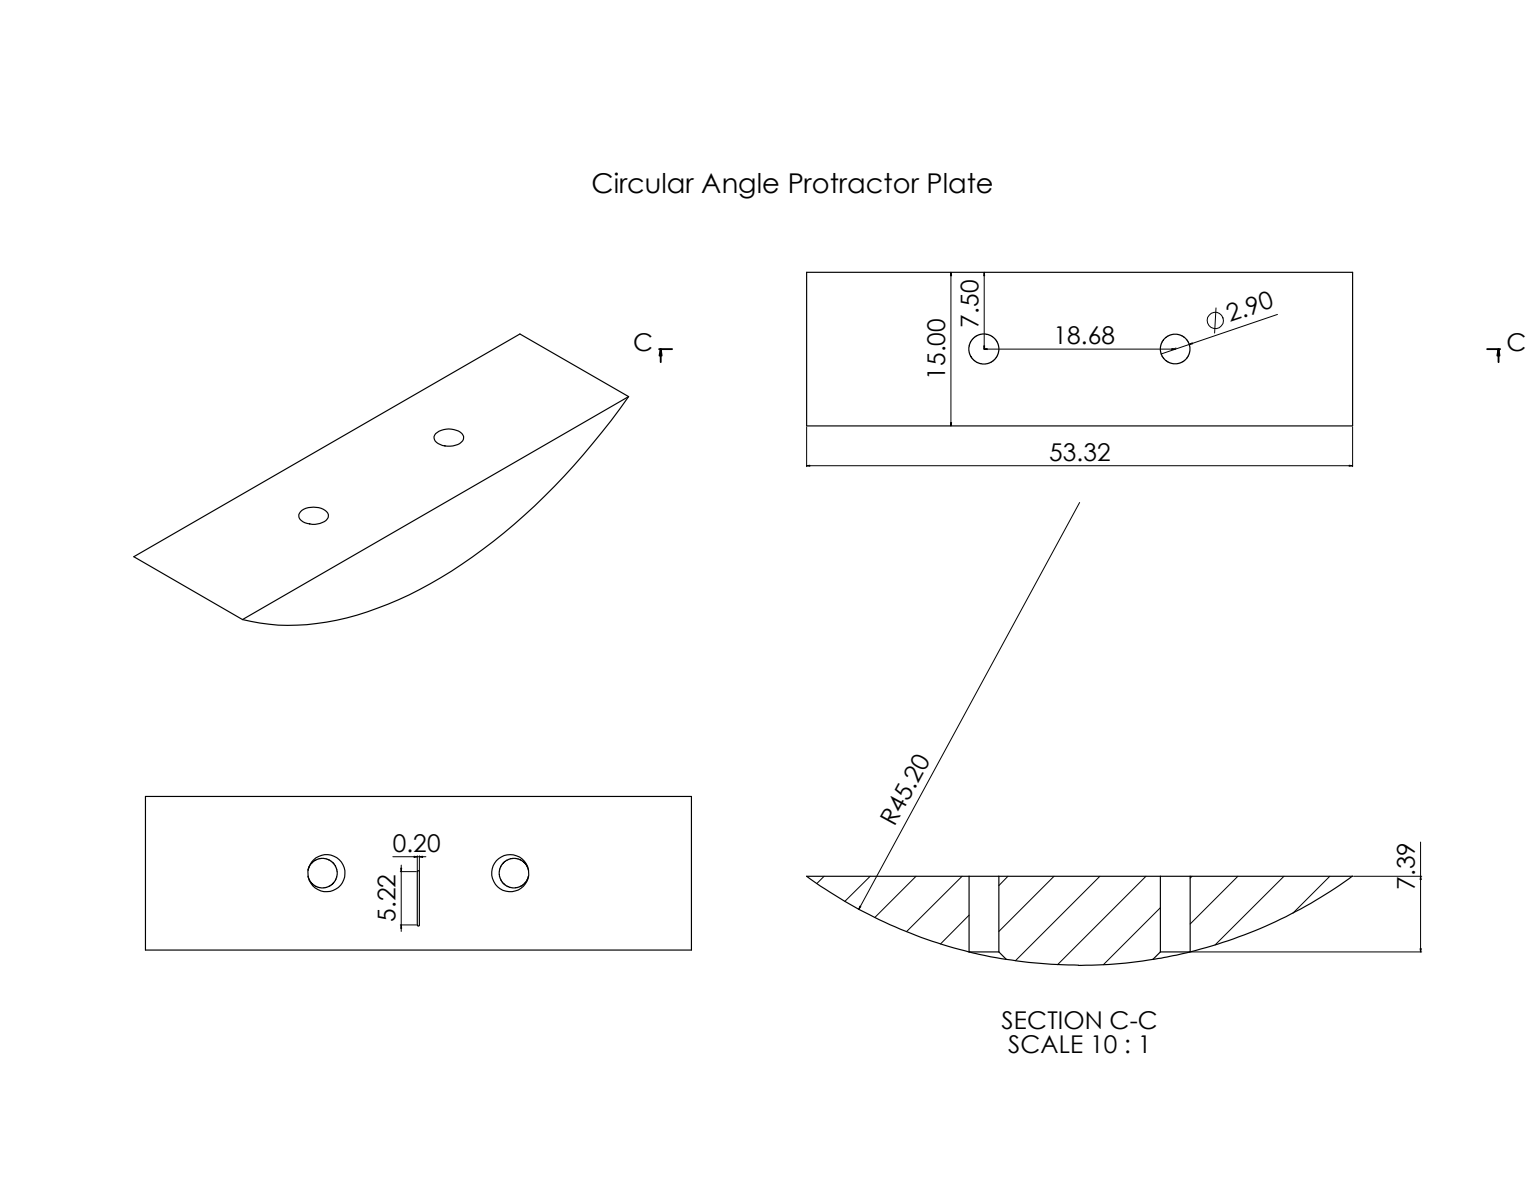
ISO-10303-21;
HEADER;
FILE_DESCRIPTION (('STEP AP214'),
    '1' );
FILE_NAME ('Circular Angle Protractor Plate.step',
    '2026-10-24T22:31:37',
    ( '' ),
    ( '' ),
    'SwSTEP 2.0',
    'SolidWorks 2025',
    '' );
FILE_SCHEMA (( 'AUTOMOTIVE_DESIGN' ));
ENDSEC;

DATA;
#164=CARTESIAN_POINT ( 'NONE',  ( -31.31952861460583648, 96.88699691338099740, 44.45098699770857564 ) ) ;
#634=B_SPLINE_CURVE_WITH_KNOTS ( 'NONE', 3,
 ( #30232, #48312, #32606, #86869, #60608, #52525 ),
 .UNSPECIFIED., .F., .F.,
 ( 4, 2, 4 ),
 ( 0.0003203576572402824438, 0.0005551992086451969666, 0.0007900407600501114895 ),
 .UNSPECIFIED. ) ;
#730=CIRCLE ( 'NONE', #57349, 1.449999999999993072 ) ;
#857=ORIENTED_EDGE ( 'NONE', *, *, #39122, .T. ) ;
#893=( NAMED_UNIT ( * ) PLANE_ANGLE_UNIT ( ) SI_UNIT ( $, .RADIAN. ) );
#992=CARTESIAN_POINT ( 'NONE',  ( -30.47963256238546492, 93.39033706315194650, 44.25085353260880794 ) ) ;
#1024=CONICAL_SURFACE ( 'NONE', #73855, 2.749999999999999112, 0.7853981633974463916 ) ;
#1224=( GEOMETRIC_REPRESENTATION_CONTEXT ( 3 ) GLOBAL_UNCERTAINTY_ASSIGNED_CONTEXT ( ( #85922 ) ) GLOBAL_UNIT_ASSIGNED_CONTEXT ( ( #100216, #893, #55077 ) ) REPRESENTATION_CONTEXT ( 'NONE', 'WORKASPACE' ) );
#1578=VERTEX_POINT ( 'NONE', #33085 ) ;
#2059=EDGE_CURVE ( 'NONE', #67256, #32333, #54564, .T. ) ;
#2273=ORIENTED_EDGE ( 'NONE', *, *, #12991, .T. ) ;
#3183=VECTOR ( 'NONE', #74444, 1000.000000000000000 ) ;
#3234=VERTEX_POINT ( 'NONE', #63225 ) ;
#3354=ADVANCED_FACE ( 'NONE', ( #93158, #47025, #11548, #50029 ), #89577, .T. ) ;
#3695=FACE_OUTER_BOUND ( 'NONE', #33468, .T. ) ;
#3766=ORIENTED_EDGE ( 'NONE', *, *, #38014, .F. ) ;
#4089=VERTEX_POINT ( 'NONE', #49422 ) ;
#4404=B_SPLINE_CURVE_WITH_KNOTS ( 'NONE', 3,
 ( #54876, #32587, #69082, #92914, #93426, #63485 ),
 .UNSPECIFIED., .F., .F.,
 ( 4, 2, 4 ),
 ( 0.006526230984275955063, 0.006760533473033110939, 0.006994835961790266815 ),
 .UNSPECIFIED. ) ;
#4502=CARTESIAN_POINT ( 'NONE',  ( -20.87573318553691593, 95.07663899570583510, 45.19945584158065799 ) ) ;
#4742=VERTEX_POINT ( 'NONE', #96901 ) ;
#4801=DIRECTION ( 'NONE',  ( 0.000000000000000000, -0.000000000000000000, 1.000000000000000000 ) ) ;
#4942=DIRECTION ( 'NONE',  ( 0.5000000000000012212, -0.8660254037844379305, -0.000000000000000000 ) ) ;
#5180=APPLICATION_CONTEXT ( 'automotive_design' ) ;
#5593=ADVANCED_FACE ( 'NONE', ( #3695 ), #78121, .F. ) ;
#5598=CARTESIAN_POINT ( 'NONE',  ( -29.38832164612380637, 94.71097215053278262, 44.55472784766640615 ) ) ;
#5830=CARTESIAN_POINT ( 'NONE',  ( -23.41475416096364981, 99.76909336696888886, 45.19938842315524852 ) ) ;
#6266=CARTESIAN_POINT ( 'NONE',  ( -32.97299853046111195, 95.39863959553431982, 43.99458562601660816 ) ) ;
#6331=CARTESIAN_POINT ( 'NONE',  ( -23.56828086056981064, 99.64628362023964314, 45.19937630303414977 ) ) ;
#6701=DIRECTION ( 'NONE',  ( 0.5000000000000012212, -0.8660254037844380415, -0.000000000000000000 ) ) ;
#6733=EDGE_CURVE ( 'NONE', #87881, #36461, #26570, .T. ) ;
#6960=ORIENTED_EDGE ( 'NONE', *, *, #89379, .T. ) ;
#7674=ORIENTED_EDGE ( 'NONE', *, *, #67129, .T. ) ;
#7748=ORIENTED_EDGE ( 'NONE', *, *, #38014, .T. ) ;
#8007=AXIS2_PLACEMENT_3D ( 'NONE', #31791, #22335, #47010 ) ;
#8055=ADVANCED_FACE ( 'NONE', ( #24452 ), #39126, .F. ) ;
#8121=CARTESIAN_POINT ( 'NONE',  ( -17.43116445825134164, 103.7197590629589712, 44.61401193002000554 ) ) ;
#8132=ORIENTED_EDGE ( 'NONE', *, *, #33889, .T. ) ;
#9002=ADVANCED_FACE ( 'NONE', ( #62292 ), #59933, .F. ) ;
#9449=CARTESIAN_POINT ( 'NONE',  ( -31.49356256989596758, 94.88921800892812541, 43.89948692389422291 ) ) ;
#9508=CARTESIAN_POINT ( 'NONE',  ( -28.74356256989596758, 94.88921800892812541, 45.19948692389422717 ) ) ;
#9555=CARTESIAN_POINT ( 'NONE',  ( -30.04356256989597185, 94.88921800892812541, 45.19948692389422717 ) ) ;
#9631=DIRECTION ( 'NONE',  ( 1.000000000000000000, 0.000000000000000000, -0.000000000000000000 ) ) ;
#9946=ORIENTED_EDGE ( 'NONE', *, *, #31896, .T. ) ;
#10277=CARTESIAN_POINT ( 'NONE',  ( -27.15312891409035601, 106.0554225863516109, 0.000000000000000000 ) ) ;
#10394=ADVANCED_FACE ( 'NONE', ( #96530 ), #92169, .F. ) ;
#10459=ORIENTED_EDGE ( 'NONE', *, *, #63681, .F. ) ;
#10513=EDGE_CURVE ( 'NONE', #3234, #18286, #87369, .T. ) ;
#10739=CARTESIAN_POINT ( 'NONE',  ( -32.70869837084711662, 94.07384053862010376, 43.88975835780059498 ) ) ;
#11221=CIRCLE ( 'NONE', #24134, 1.449999999999993072 ) ;
#11254=DIRECTION ( 'NONE',  ( -0.5000000000000013323, 0.8660254037844380415, -0.000000000000000000 ) ) ;
#11483=EDGE_CURVE ( 'NONE', #94973, #64873, #72785, .T. ) ;
#11548=FACE_BOUND ( 'NONE', #36641, .T. ) ;
#11932=DIRECTION ( 'NONE',  ( -0.000000000000000000, -0.000000000000000000, 1.000000000000000000 ) ) ;
#12100=CARTESIAN_POINT ( 'NONE',  ( -4.065086259125790136, 119.3853102282570120, 36.50000000000000000 ) ) ;
#12128=EDGE_CURVE ( 'NONE', #34739, #4742, #40374, .T. ) ;
#12490=ORIENTED_EDGE ( 'NONE', *, *, #73839, .F. ) ;
#12829=CARTESIAN_POINT ( 'NONE',  ( -32.94356256989595977, 94.88921800892812541, 43.89948692389422291 ) ) ;
#12963=CARTESIAN_POINT ( 'NONE',  ( -23.57869195597365319, 99.67400356242829673, 45.19938701403189896 ) ) ;
#12991=EDGE_CURVE ( 'NONE', #28157, #34739, #36053, .T. ) ;
#13370=DIRECTION ( 'NONE',  ( 1.000000000000000000, 0.000000000000000000, 0.000000000000000000 ) ) ;
#13586=DIRECTION ( 'NONE',  ( 1.000000000000000000, 0.000000000000000000, 0.000000000000000000 ) ) ;
#13614=CARTESIAN_POINT ( 'NONE',  ( -20.77255224845912451, 95.18466417500319210, 45.19939659820781230 ) ) ;
#13932=CARTESIAN_POINT ( 'NONE',  ( -23.49900916367506198, 99.79204404934422712, 45.19947629006753687 ) ) ;
#14107=CARTESIAN_POINT ( 'NONE',  ( -20.77265562100329532, 95.16204261274404530, 45.19941863730353049 ) ) ;
#14393=VECTOR ( 'NONE', #66956, 1000.000000000000227 ) ;
#14436=CARTESIAN_POINT ( 'NONE',  ( -23.53063603519568048, 99.78015757744582004, 45.19948828869558355 ) ) ;
#14500=CONICAL_SURFACE ( 'NONE', #25803, 2.749999999999999112, 0.7853981633974469467 ) ;
#14548=ORIENTED_EDGE ( 'NONE', *, *, #29889, .T. ) ;
#14567=ORIENTED_EDGE ( 'NONE', *, *, #80039, .T. ) ;
#14574=EDGE_LOOP ( 'NONE', ( #42344, #84005, #99466 ) ) ;
#14607=CARTESIAN_POINT ( 'NONE',  ( -20.90861557574503848, 95.08343395685160715, 45.19941947175312436 ) ) ;
#14848=CARTESIAN_POINT ( 'NONE',  ( -15.28083007106358693, 105.8318407428233030, 44.04068696433692054 ) ) ;
#14913=CARTESIAN_POINT ( 'NONE',  ( -23.56906976425110400, 99.73991939959820741, 45.19945594742419104 ) ) ;
#15191=CARTESIAN_POINT ( 'NONE',  ( -13.95037114427627500, 103.3647202663174056, 44.05931802377998707 ) ) ;
#15209=CARTESIAN_POINT ( 'NONE',  ( -17.43550054826663498, 104.2312461070085021, 44.57229221387615326 ) ) ;
#15354=CARTESIAN_POINT ( 'NONE',  ( 0.000000000000000000, 0.000000000000000000, 0.000000000000000000 ) ) ;
#15532=DIRECTION ( 'NONE',  ( 1.000000000000000000, 0.000000000000000000, 0.000000000000000000 ) ) ;
#15676=CARTESIAN_POINT ( 'NONE',  ( -31.52638293593248164, 93.28895303089220192, 44.04053121186087338 ) ) ;
#15694=FACE_BOUND ( 'NONE', #45535, .T. ) ;
#15696=CARTESIAN_POINT ( 'NONE',  ( -16.11791840453430780, 102.2811357711566131, 44.54428794602774389 ) ) ;
#15849=CARTESIAN_POINT ( 'NONE',  ( -29.49634561128635468, 95.76491754085807884, 44.62645301900288075 ) ) ;
#16389=ORIENTED_EDGE ( 'NONE', *, *, #62910, .T. ) ;
#16591=CARTESIAN_POINT ( 'NONE',  ( -50.24117156905492720, 92.72553494444620981, 36.50000000000000000 ) ) ;
#16597=DIRECTION ( 'NONE',  ( 1.000000000000000000, 0.000000000000000000, 0.000000000000000000 ) ) ;
#16845=DIRECTION ( 'NONE',  ( 1.000000000000000000, 0.000000000000000000, 0.000000000000000000 ) ) ;
#17040=EDGE_CURVE ( 'NONE', #36797, #52552, #76756, .T. ) ;
#17072=CIRCLE ( 'NONE', #62395, 45.19948692389424139 ) ;
#17190=ORIENTED_EDGE ( 'NONE', *, *, #10513, .T. ) ;
#17249=VECTOR ( 'NONE', #70280, 1000.000000000000000 ) ;
#17416=CARTESIAN_POINT ( 'NONE',  ( -31.49356256989596758, 94.88921800892812541, 45.19948692389422717 ) ) ;
#17441=AXIS2_PLACEMENT_3D ( 'NONE', #52341, #83283, #13370 ) ;
#17526=ORIENTED_EDGE ( 'NONE', *, *, #75938, .T. ) ;
#17540=VECTOR ( 'NONE', #52128, 1000.000000000000000 ) ;
#17603=B_SPLINE_CURVE_WITH_KNOTS ( 'NONE', 3,
 ( #90978, #83366, #52922, #5830, #21538, #52421, #67624, #30123, #99049, #37710, #59511, #13932, #45317, #68618, #14436, #36223, #44811, #91461, #61005, #14913, #67125, #36720, #53416, #59005, #98049, #12963, #75748, #76252, #99541, #6331, #68121 ),
 .UNSPECIFIED., .F., .F.,
 ( 4, 3, 3, 3, 3, 3, 3, 3, 3, 3, 4 ),
 ( 0.000000000000000000, 3.357709145156238112E-05, 6.715417940116638184E-05, 0.0001007313198657320137, 0.0001343084960840525556, 0.0001678856156954656629, 0.0002014626747008688135, 0.0002350397637044835341, 0.0002686169264846348381, 0.0003021940916574198136, 0.0003125816342522854925 ),
 .UNSPECIFIED. ) ;
#17632=ORIENTED_EDGE ( 'NONE', *, *, #17040, .F. ) ;
#17761=AXIS2_PLACEMENT_3D ( 'NONE', #9449, #70741, #78864 ) ;
#17958=EDGE_CURVE ( 'NONE', #36461, #36797, #55136, .T. ) ;
#18072=DIRECTION ( 'NONE',  ( 0.000000000000000000, -0.000000000000000000, 1.000000000000000000 ) ) ;
#18176=AXIS2_PLACEMENT_3D ( 'NONE', #42892, #4942, #81464 ) ;
#18286=VERTEX_POINT ( 'NONE', #19836 ) ;
#18380=FACE_OUTER_BOUND ( 'NONE', #96719, .T. ) ;
#19111=CARTESIAN_POINT ( 'NONE',  ( -14.45063460946529155, 102.6502293776574390, 44.23345500514351869 ) ) ;
#19161=LINE ( 'NONE', #9555, #51387 ) ;
#19275=ORIENTED_EDGE ( 'NONE', *, *, #74132, .F. ) ;
#19559=ORIENTED_EDGE ( 'NONE', *, *, #39122, .F. ) ;
#19836=CARTESIAN_POINT ( 'NONE',  ( -30.04356256989597185, 94.88921800892812541, 36.50000000000000000 ) ) ;
#20094=EDGE_CURVE ( 'NONE', #91664, #32333, #33062, .T. ) ;
#20164=ORIENTED_EDGE ( 'NONE', *, *, #54513, .T. ) ;
#20720=CARTESIAN_POINT ( 'NONE',  ( -20.77345734792011456, 95.19581990215550604, 45.19938701403189896 ) ) ;
#21018=DIRECTION ( 'NONE',  ( 0.5000000000000012212, -0.8660254037844379305, -0.000000000000000000 ) ) ;
#21216=CARTESIAN_POINT ( 'NONE',  ( -20.92890603600389099, 95.09343599062782459, 45.19939615752831230 ) ) ;
#21404=ADVANCED_FACE ( 'NONE', ( #29286 ), #21966, .F. ) ;
#21421=AXIS2_PLACEMENT_3D ( 'NONE', #51780, #82720, #67459 ) ;
#21463=CARTESIAN_POINT ( 'NONE',  ( -17.14183914111196927, 105.0694402252967024, 44.45399967932692675 ) ) ;
#21538=CARTESIAN_POINT ( 'NONE',  ( -23.42324326788986610, 99.77638747395597818, 45.19939615752831230 ) ) ;
#21548=ORIENTED_EDGE ( 'NONE', *, *, #23427, .T. ) ;
#21703=CARTESIAN_POINT ( 'NONE',  ( -20.78934165772523812, 95.12062749311181165, 45.19946569820528737 ) ) ;
#21731=CARTESIAN_POINT ( 'NONE',  ( -18.06269525828470890, 104.2312461070085021, 45.19948692389422717 ) ) ;
#21955=CARTESIAN_POINT ( 'NONE',  ( -16.48692306231661320, 105.6553858747601424, 44.28718864051150206 ) ) ;
#21966=CONICAL_SURFACE ( 'NONE', #93154, 2.749999999999999112, 0.7853981633974463916 ) ;
#22200=CARTESIAN_POINT ( 'NONE',  ( -20.94588425035955837, 95.10802420503439691, 45.19938068878172288 ) ) ;
#22335=DIRECTION ( 'NONE',  ( 0.5000000000000012212, -0.8660254037844379305, 0.000000000000000000 ) ) ;
#22463=CARTESIAN_POINT ( 'NONE',  ( -29.75479735258813108, 96.20417995190686611, 44.62577945616610009 ) ) ;
#22670=EDGE_LOOP ( 'NONE', ( #48559, #38821 ) ) ;
#22689=CARTESIAN_POINT ( 'NONE',  ( -32.97666635132488011, 94.88921800892812541, 43.93259070532314325 ) ) ;
#22707=CARTESIAN_POINT ( 'NONE',  ( -20.78227252765418953, 95.22040553774976956, 45.19937671356586861 ) ) ;
#22726=CARTESIAN_POINT ( 'NONE',  ( -13.99899119970020145, 104.8759001898749688, 43.88975813191157016 ) ) ;
#22804=EDGE_LOOP ( 'NONE', ( #43817, #72902, #87127, #30741 ) ) ;
#22812=CARTESIAN_POINT ( 'NONE',  ( -13.80441806700167007, 103.9794969232740272, 43.95776411517724824 ) ) ;
#22914=ADVANCED_FACE ( 'NONE', ( #93461 ), #24014, .F. ) ;
#22929=LINE ( 'NONE', #69536, #59476 ) ;
#23297=CARTESIAN_POINT ( 'NONE',  ( -17.25743208833890208, 103.2403577256391998, 44.62839627432005329 ) ) ;
#23427=EDGE_CURVE ( 'NONE', #18286, #3234, #83624, .T. ) ;
#23457=DIRECTION ( 'NONE',  ( 1.000000000000000000, 0.000000000000000000, 0.000000000000000000 ) ) ;
#23779=CARTESIAN_POINT ( 'NONE',  ( -31.34720201560244845, 93.26289111443594493, 44.07321716645989085 ) ) ;
#24014=CYLINDRICAL_SURFACE ( 'NONE', #68886, 1.449999999999993072 ) ;
#24134=AXIS2_PLACEMENT_3D ( 'NONE', #35210, #11932, #81362 ) ;
#24314=CARTESIAN_POINT ( 'NONE',  ( -17.31098718113245027, 103.3584764561434639, 44.62636701040934639 ) ) ;
#24324=DIRECTION ( 'NONE',  ( 1.000000000000000000, 0.000000000000000000, 0.000000000000000000 ) ) ;
#24327=ORIENTED_EDGE ( 'NONE', *, *, #6733, .F. ) ;
#24452=FACE_OUTER_BOUND ( 'NONE', #64344, .T. ) ;
#24742=VECTOR ( 'NONE', #49001, 1000.000000000000000 ) ;
#24778=CARTESIAN_POINT ( 'NONE',  ( -32.32800653043278061, 93.66491217184130846, 43.92044614505844891 ) ) ;
#25526=DIRECTION ( 'NONE',  ( 1.000000000000000000, 0.000000000000000000, 0.000000000000000000 ) ) ;
#25803=AXIS2_PLACEMENT_3D ( 'NONE', #36665, #65583, #73696 ) ;
#25945=CARTESIAN_POINT ( 'NONE',  ( -27.15312891409035601, 106.0554225863516109, 0.000000000000000000 ) ) ;
#25985=DIRECTION ( 'NONE',  ( 0.8660254037844379305, 0.5000000000000012212, 0.000000000000000000 ) ) ;
#26378=ORIENTED_EDGE ( 'NONE', *, *, #12991, .F. ) ;
#26439=DIRECTION ( 'NONE',  ( 0.8660254037844378194, 0.5000000000000013323, 0.000000000000000000 ) ) ;
#26520=PRODUCT ( 'Circular Angle Protractor Plate', 'Circular Angle Protractor Plate', '', ( #84692 ) ) ;
#26570=LINE ( 'NONE', #73670, #83871 ) ;
#27015=LINE ( 'NONE', #27520, #46114 ) ;
#27090=CARTESIAN_POINT ( 'NONE',  ( -32.85588310213878316, 95.75574514201873910, 44.05931881766424141 ) ) ;
#27520=CARTESIAN_POINT ( 'NONE',  ( -13.86269525828471849, 104.2312461070085021, 45.19948692389422717 ) ) ;
#27615=CYLINDRICAL_SURFACE ( 'NONE', #66836, 45.19948692389423428 ) ;
#28157=VERTEX_POINT ( 'NONE', #12100 ) ;
#28294=CARTESIAN_POINT ( 'NONE',  ( -20.91904052551286597, 95.08750694953491234, 45.19940739266792207 ) ) ;
#28805=CARTESIAN_POINT ( 'NONE',  ( -20.77164714902255582, 95.17350844815184985, 45.19940618238346275 ) ) ;
#28949=CARTESIAN_POINT ( 'NONE',  ( -13.86269525828471672, 104.2312461070085021, 43.89948692389422291 ) ) ;
#29093=DIRECTION ( 'NONE',  ( -0.000000000000000000, -0.000000000000000000, 1.000000000000000000 ) ) ;
#29160=ORIENTED_EDGE ( 'NONE', *, *, #75790, .F. ) ;
#29286=FACE_OUTER_BOUND ( 'NONE', #31222, .T. ) ;
#29311=CARTESIAN_POINT ( 'NONE',  ( -20.84245520245646333, 95.08111133751313560, 45.19948159324908943 ) ) ;
#29552=ADVANCED_BREP_SHAPE_REPRESENTATION ( '', ( #76389, #68784 ), #70444 ) ;
#29690=CARTESIAN_POINT ( 'NONE',  ( -32.57773935851065517, 93.92637809958223727, 43.89948692389421581 ) ) ;
#29889=EDGE_CURVE ( 'NONE', #94973, #1578, #40371, .T. ) ;
#30057=CARTESIAN_POINT ( 'NONE',  ( -32.67881874348327642, 96.08878909247250988, 44.13137598596502187 ) ) ;
#30069=CARTESIAN_POINT ( 'NONE',  ( -31.49356256989596758, 94.88921800892812541, 36.50000000000000000 ) ) ;
#30123=CARTESIAN_POINT ( 'NONE',  ( -23.45395869395431632, 99.79046250668140772, 45.19943155085691444 ) ) ;
#30179=LINE ( 'NONE', #89189, #3183 ) ;
#30232=CARTESIAN_POINT ( 'NONE',  ( -32.86949478547433046, 94.43171332246730287, 43.89948692389422291 ) ) ;
#30274=CIRCLE ( 'NONE', #54546, 1.449999999999993072 ) ;
#30513=EDGE_CURVE ( 'NONE', #62347, #4089, #77202, .T. ) ;
#30559=CARTESIAN_POINT ( 'NONE',  ( -14.22851846967002487, 105.1940860163543476, 43.89948692389422291 ) ) ;
#30574=CARTESIAN_POINT ( 'NONE',  ( -31.49356256989596758, 94.88921800892812541, 43.89948692389422291 ) ) ;
#30661=AXIS2_PLACEMENT_3D ( 'NONE', #44267, #29093, #82340 ) ;
#30740=VERTEX_POINT ( 'NONE', #29690 ) ;
#30741=ORIENTED_EDGE ( 'NONE', *, *, #12128, .T. ) ;
#30762=FACE_OUTER_BOUND ( 'NONE', #53261, .T. ) ;
#30889=CARTESIAN_POINT ( 'NONE',  ( -29.89096190292416821, 93.77824852085353768, 44.39154330738892895 ) ) ;
#30908=CARTESIAN_POINT ( 'NONE',  ( -17.46030756596911360, 103.9795007202521475, 44.59709923157863187 ) ) ;
#31044=CARTESIAN_POINT ( 'NONE',  ( -17.23615303860155379, 104.9140057318794703, 44.48293588312308344 ) ) ;
#31051=CARTESIAN_POINT ( 'NONE',  ( -30.34080891622166121, 96.68806665343463180, 44.58230547404211563 ) ) ;
#31222=EDGE_LOOP ( 'NONE', ( #29160, #7748, #53931, #62389 ) ) ;
#31389=AXIS2_PLACEMENT_3D ( 'NONE', #10277, #33067, #25985 ) ;
#31521=DIRECTION ( 'NONE',  ( -0.8660254037844378194, -0.5000000000000013323, -0.000000000000000000 ) ) ;
#31791=CARTESIAN_POINT ( 'NONE',  ( -19.65312891409034179, 93.06504152958504505, 0.000000000000000000 ) ) ;
#31872=CARTESIAN_POINT ( 'NONE',  ( -30.81750703737776220, 93.28907056446753643, 44.17799681287748115 ) ) ;
#31895=CARTESIAN_POINT ( 'NONE',  ( -16.58100052909938071, 102.4826666393443304, 44.59494843596851155 ) ) ;
#31896=EDGE_CURVE ( 'NONE', #30740, #63497, #70158, .T. ) ;
#31905=DIRECTION ( 'NONE',  ( -0.000000000000000000, -0.000000000000000000, 1.000000000000000000 ) ) ;
#32333=VERTEX_POINT ( 'NONE', #98726 ) ;
#32587=CARTESIAN_POINT ( 'NONE',  ( -13.90914858307771063, 104.6155556099271280, 43.90259622397829986 ) ) ;
#32606=CARTESIAN_POINT ( 'NONE',  ( -32.91998363024201524, 94.57991847588093037, 43.90692951987065129 ) ) ;
#33062=B_SPLINE_CURVE_WITH_KNOTS ( 'NONE', 3,
 ( #44747, #50866, #6266, #27090, #50370, #30057, #38654, #68061, #69558, #93397, #68556, #99482, #164, #47252, #46234, #39133, #60949, #31051, #77159, #91907, #37162, #22463, #98984, #54850, #15849, #53358, #46757, #61938, #61451, #92402 ),
 .UNSPECIFIED., .F., .F.,
 ( 4, 2, 2, 2, 2, 2, 2, 2, 2, 2, 2, 2, 2, 2, 4 ),
 ( 0.0007900407600501114895, 0.001551840822610036589, 0.001932740853890018654, 0.002313640885170001153, 0.003075440947729968753, 0.003456340979009963395, 0.003837241010289958038, 0.004218141041569941838, 0.004599041072849926505, 0.004979941104129911172, 0.005360841135409894972, 0.005741741166689878773, 0.006122641197969864307, 0.006503541229249848107, 0.006884441260529831907 ),
 .UNSPECIFIED. ) ;
#33067=DIRECTION ( 'NONE',  ( 0.5000000000000012212, -0.8660254037844379305, 0.000000000000000000 ) ) ;
#33085=CARTESIAN_POINT ( 'NONE',  ( -16.76269525828470464, 104.2312461070085021, 43.89948692389422291 ) ) ;
#33206=CARTESIAN_POINT ( 'NONE',  ( -15.31269525828471068, 104.2312461070085021, 36.50000000000000000 ) ) ;
#33213=ORIENTED_EDGE ( 'NONE', *, *, #97554, .T. ) ;
#33391=AXIS2_PLACEMENT_3D ( 'NONE', #91101, #68250, #15532 ) ;
#33468=EDGE_LOOP ( 'NONE', ( #12490, #82135, #57494 ) ) ;
#33646=ORIENTED_EDGE ( 'NONE', *, *, #88200, .F. ) ;
#33889=EDGE_CURVE ( 'NONE', #100289, #82522, #45736, .T. ) ;
#33998=ORIENTED_EDGE ( 'NONE', *, *, #63681, .T. ) ;
#34021=VERTEX_POINT ( 'NONE', #12829 ) ;
#34594=CARTESIAN_POINT ( 'NONE',  ( -16.76269525828470464, 104.2312461070085021, 36.50000000000000000 ) ) ;
#34739=VERTEX_POINT ( 'NONE', #77861 ) ;
#35210=CARTESIAN_POINT ( 'NONE',  ( -31.49356256989596758, 94.88921800892812541, 43.89948692389422291 ) ) ;
#35402=CARTESIAN_POINT ( 'NONE',  ( -20.83177028255669683, 95.08444325421659471, 45.19948689642177442 ) ) ;
#35666=CARTESIAN_POINT ( 'NONE',  ( -17.43550054826663498, 104.2312461070085021, 44.57229221387615326 ) ) ;
#35866=ORIENTED_EDGE ( 'NONE', *, *, #23427, .F. ) ;
#36053=LINE ( 'NONE', #44639, #14393 ) ;
#36149=CLOSED_SHELL ( 'NONE', ( #5593, #58964, #22914, #21404, #10394, #9002, #3354, #93783, #48551, #43723, #72414, #47780, #49821, #8055, #72966 ) ) ;
#36223=CARTESIAN_POINT ( 'NONE',  ( -23.53961575219861402, 99.77347671786461092, 45.19948544083312214 ) ) ;
#36329=DIRECTION ( 'NONE',  ( 1.000000000000000000, 0.000000000000000000, 0.000000000000000000 ) ) ;
#36461=VERTEX_POINT ( 'NONE', #86048 ) ;
#36641=EDGE_LOOP ( 'NONE', ( #6960, #52750, #7674, #9946 ) ) ;
#36665=CARTESIAN_POINT ( 'NONE',  ( -31.49356256989596758, 94.88921800892812541, 45.19948692389422717 ) ) ;
#36720=CARTESIAN_POINT ( 'NONE',  ( -23.57665515266768352, 99.71860730699962971, 45.19943101769310090 ) ) ;
#36797=VERTEX_POINT ( 'NONE', #86097 ) ;
#36895=CARTESIAN_POINT ( 'NONE',  ( -20.85314014021869866, 95.07777941523956144, 45.19947629006753687 ) ) ;
#36915=CARTESIAN_POINT ( 'NONE',  ( -13.93676304270635136, 104.6887507934693105, 43.89948692389422291 ) ) ;
#37091=CARTESIAN_POINT ( 'NONE',  ( -13.86269525828471849, 104.2312461070085021, 36.50000000000000000 ) ) ;
#37111=ORIENTED_EDGE ( 'NONE', *, *, #97554, .F. ) ;
#37147=EDGE_LOOP ( 'NONE', ( #58527, #33213, #72176, #55276, #14567, #10459 ) ) ;
#37162=CARTESIAN_POINT ( 'NONE',  ( -29.92656730811346222, 96.39204771392240900, 44.61692575031640473 ) ) ;
#37420=LINE ( 'NONE', #76926, #17540 ) ;
#37474=CARTESIAN_POINT ( 'NONE',  ( -29.43245964505113932, 94.53574275318644027, 44.53316583206422763 ) ) ;
#37710=CARTESIAN_POINT ( 'NONE',  ( -23.47641611835684117, 99.79318446887796767, 45.19945584158065799 ) ) ;
#38014=EDGE_CURVE ( 'NONE', #1578, #82522, #60206, .T. ) ;
#38646=CARTESIAN_POINT ( 'NONE',  ( -16.78138373794034877, 105.4614945587019577, 44.35755392706056455 ) ) ;
#38654=CARTESIAN_POINT ( 'NONE',  ( -32.60591808846487538, 96.18968631316256790, 44.15639294459641917 ) ) ;
#38745=CARTESIAN_POINT ( 'NONE',  ( -27.06652637371191616, 106.1054225863516081, 45.19937630303414267 ) ) ;
#38821=ORIENTED_EDGE ( 'NONE', *, *, #11483, .T. ) ;
#39122=EDGE_CURVE ( 'NONE', #56639, #1578, #96840, .T. ) ;
#39126=CYLINDRICAL_SURFACE ( 'NONE', #98308, 1.449999999999993072 ) ;
#39133=CARTESIAN_POINT ( 'NONE',  ( -30.69451156873374487, 96.82744408686065185, 44.54218732323495544 ) ) ;
#39481=CARTESIAN_POINT ( 'NONE',  ( -15.86348812680012799, 102.2296172668195737, 44.51064192688916421 ) ) ;
#39985=CARTESIAN_POINT ( 'NONE',  ( -14.20026547392215477, 102.9308592454766966, 44.15637032012459429 ) ) ;
#40371=LINE ( 'NONE', #86062, #17249 ) ;
#40374=LINE ( 'NONE', #16591, #40392 ) ;
#40392=VECTOR ( 'NONE', #93630, 999.9999999999998863 ) ;
#40809=CARTESIAN_POINT ( 'NONE',  ( -32.94356256989595977, 94.88921800892812541, 45.19948692389422717 ) ) ;
#41544=EDGE_CURVE ( 'NONE', #4742, #43464, #89838, .T. ) ;
#41823=DIRECTION ( 'NONE',  ( -0.000000000000000000, -0.000000000000000000, 1.000000000000000000 ) ) ;
#42344=ORIENTED_EDGE ( 'NONE', *, *, #2059, .F. ) ;
#42892=CARTESIAN_POINT ( 'NONE',  ( -27.15312891409035601, 106.0554225863516109, 0.000000000000000000 ) ) ;
#43235=CARTESIAN_POINT ( 'NONE',  ( -15.31269525828471068, 104.2312461070085021, 43.89948692389422291 ) ) ;
#43464=VERTEX_POINT ( 'NONE', #93569 ) ;
#43723=ADVANCED_FACE ( 'NONE', ( #18380 ), #48271, .F. ) ;
#43817=ORIENTED_EDGE ( 'NONE', *, *, #41544, .T. ) ;
#44267=CARTESIAN_POINT ( 'NONE',  ( -15.31269525828471068, 104.2312461070085021, 45.19948692389422717 ) ) ;
#44268=DIRECTION ( 'NONE',  ( 1.000000000000000000, 0.000000000000000000, 0.000000000000000000 ) ) ;
#44355=ORIENTED_EDGE ( 'NONE', *, *, #50440, .F. ) ;
#44639=CARTESIAN_POINT ( 'NONE',  ( -50.24117156905492720, 92.72553494444620981, 36.50000000000000000 ) ) ;
#44747=CARTESIAN_POINT ( 'NONE',  ( -32.97666635132488011, 94.88921800892812541, 43.93259070532314325 ) ) ;
#44811=CARTESIAN_POINT ( 'NONE',  ( -23.54859545362356243, 99.76679586987334858, 45.19948259297560611 ) ) ;
#45317=CARTESIAN_POINT ( 'NONE',  ( -23.50969410143729377, 99.78871212707066718, 45.19948159324908943 ) ) ;
#45485=CARTESIAN_POINT ( 'NONE',  ( -20.89819060993944078, 95.07936095790239506, 45.19943155085691444 ) ) ;
#45535=EDGE_LOOP ( 'NONE', ( #21548, #17190 ) ) ;
#45734=CARTESIAN_POINT ( 'NONE',  ( -14.34210371876190315, 105.3327122335069816, 43.90660993338509144 ) ) ;
#45736=B_SPLINE_CURVE_WITH_KNOTS ( 'NONE', 3,
 ( #92263, #22812, #53692, #15191, #69899, #62798, #39985, #19111, #93242, #54184, #70922, #88545, #57572, #39481, #15696, #31895, #93754, #80434, #94248, #23297, #24314, #8121, #30908, #78527 ),
 .UNSPECIFIED., .F., .F.,
 ( 4, 2, 2, 2, 2, 2, 2, 2, 2, 2, 2, 4 ),
 ( 0.006994835961790266815, 0.007754851833055070344, 0.008134859768687469073, 0.008514867704319870403, 0.009274883575584667861, 0.009654891511217062253, 0.01003489944684945491, 0.01079491531811423849, 0.01155493118937902207, 0.01193493912501142687, 0.01231494706064382993, 0.01307496293190867249 ),
 .UNSPECIFIED. ) ;
#46075=EDGE_CURVE ( 'NONE', #64873, #94973, #730, .T. ) ;
#46114=VECTOR ( 'NONE', #97424, 1000.000000000000000 ) ;
#46227=CARTESIAN_POINT ( 'NONE',  ( -17.37321732699747656, 104.5861979058573752, 44.53294705236607598 ) ) ;
#46234=CARTESIAN_POINT ( 'NONE',  ( -30.94311057985214575, 96.87776860595468520, 44.50898273599062804 ) ) ;
#46571=CARTESIAN_POINT ( 'NONE',  ( -32.03049420854435425, 93.46753386908051198, 43.95878507283718761 ) ) ;
#46590=CARTESIAN_POINT ( 'NONE',  ( -50.24117156905492720, 92.72553494444620981, 36.50000000000000000 ) ) ;
#46757=CARTESIAN_POINT ( 'NONE',  ( -29.38772878418747325, 95.39667460785805986, 44.61190340104155894 ) ) ;
#46988=EDGE_CURVE ( 'NONE', #64873, #62347, #27015, .T. ) ;
#47010=DIRECTION ( 'NONE',  ( 0.8660254037844379305, 0.5000000000000012212, 0.000000000000000000 ) ) ;
#47025=FACE_BOUND ( 'NONE', #65930, .T. ) ;
#47082=CARTESIAN_POINT ( 'NONE',  ( -29.66248920917699294, 94.05350397404733087, 44.45454265775622105 ) ) ;
#47252=CARTESIAN_POINT ( 'NONE',  ( -31.06813028187898240, 96.88955183556316797, 44.49079097436682417 ) ) ;
#47488=CARTESIAN_POINT ( 'NONE',  ( -20.78562219458220284, 95.22657743062728741, 45.19937630303414267 ) ) ;
#47780=ADVANCED_FACE ( 'NONE', ( #51539 ), #50048, .F. ) ;
#48271=PLANE ( 'NONE',  #31389 ) ;
#48312=CARTESIAN_POINT ( 'NONE',  ( -32.89710813242851373, 94.50490555674265636, 43.90259609869470125 ) ) ;
#48472=B_SPLINE_CURVE_WITH_KNOTS ( 'NONE', 3,
 ( #52606, #92176, #22726, #36915 ),
 .UNSPECIFIED., .F., .F.,
 ( 4, 4 ),
 ( 1.636534854170084423E-17, 0.0005839710162101579682 ),
 .UNSPECIFIED. ) ;
#48490=EDGE_CURVE ( 'NONE', #34739, #28157, #17072, .T. ) ;
#48551=ADVANCED_FACE ( 'NONE', ( #15694, #55678, #93752 ), #54682, .F. ) ;
#48559=ORIENTED_EDGE ( 'NONE', *, *, #46075, .T. ) ;
#48958=ORIENTED_EDGE ( 'NONE', *, *, #29889, .F. ) ;
#49001=DIRECTION ( 'NONE',  ( 0.7071067811865465735, 0.000000000000000000, 0.7071067811865484609 ) ) ;
#49033=DIRECTION ( 'NONE',  ( 0.8660254037844380415, 0.5000000000000011102, 0.000000000000000000 ) ) ;
#49339=ORIENTED_EDGE ( 'NONE', *, *, #6733, .T. ) ;
#49422=CARTESIAN_POINT ( 'NONE',  ( -13.93676304270635136, 104.6887507934693105, 43.89948692389422291 ) ) ;
#49821=ADVANCED_FACE ( 'NONE', ( #55086 ), #1024, .F. ) ;
#50029=FACE_BOUND ( 'NONE', #74095, .T. ) ;
#50048=CYLINDRICAL_SURFACE ( 'NONE', #86695, 1.449999999999993072 ) ;
#50370=CARTESIAN_POINT ( 'NONE',  ( -32.80384426222999394, 95.87215644830973815, 44.08287417880057291 ) ) ;
#50440=EDGE_CURVE ( 'NONE', #56639, #4089, #48472, .T. ) ;
#50866=CARTESIAN_POINT ( 'NONE',  ( -33.00185145827278177, 95.14108417060988643, 43.95777581227104491 ) ) ;
#51340=DIRECTION ( 'NONE',  ( -0.000000000000000000, -0.000000000000000000, 1.000000000000000000 ) ) ;
#51387=VECTOR ( 'NONE', #95182, 1000.000000000000000 ) ;
#51539=FACE_OUTER_BOUND ( 'NONE', #58848, .T. ) ;
#51780=CARTESIAN_POINT ( 'NONE',  ( -31.49356256989596758, 94.88921800892812541, 45.19948692389422717 ) ) ;
#51809=APPLICATION_CONTEXT ( 'automotive_design' ) ;
#52124=ORIENTED_EDGE ( 'NONE', *, *, #75790, .T. ) ;
#52128=DIRECTION ( 'NONE',  ( 0.7071067811865462405, 0.000000000000000000, 0.7071067811865489050 ) ) ;
#52341=CARTESIAN_POINT ( 'NONE',  ( -15.31269525828471068, 104.2312461070085021, 45.19948692389422717 ) ) ;
#52351=CARTESIAN_POINT ( 'NONE',  ( -15.81198528973881778, 105.8575200343950229, 44.14166339942401152 ) ) ;
#52421=CARTESIAN_POINT ( 'NONE',  ( -23.43310877838089112, 99.78231651504889044, 45.19940739266792207 ) ) ;
#52525=CARTESIAN_POINT ( 'NONE',  ( -32.97666635132488011, 94.88921800892812541, 43.93259070532314325 ) ) ;
#52552=VERTEX_POINT ( 'NONE', #74414 ) ;
#52559=CARTESIAN_POINT ( 'NONE',  ( -15.31269525828471068, 104.2312461070085021, 45.19948692389422717 ) ) ;
#52606=CARTESIAN_POINT ( 'NONE',  ( -14.22851846967002487, 105.1940860163543476, 43.89948692389422291 ) ) ;
#52635=ORIENTED_EDGE ( 'NONE', *, *, #30513, .T. ) ;
#52750=ORIENTED_EDGE ( 'NONE', *, *, #20094, .T. ) ;
#52922=CARTESIAN_POINT ( 'NONE',  ( -23.40626505353419873, 99.76179925954940586, 45.19938068878172288 ) ) ;
#53067=DIRECTION ( 'NONE',  ( -0.000000000000000000, -0.000000000000000000, 1.000000000000000000 ) ) ;
#53094=CARTESIAN_POINT ( 'NONE',  ( -20.95323109343049239, 95.11688455923321328, 45.19937630303414977 ) ) ;
#53261=EDGE_LOOP ( 'NONE', ( #79814, #90626, #95456, #72674 ) ) ;
#53358=CARTESIAN_POINT ( 'NONE',  ( -29.41492724108444889, 95.52075410896856056, 44.61813138648138732 ) ) ;
#53416=CARTESIAN_POINT ( 'NONE',  ( -23.57949368289046888, 99.70778085183977169, 45.19941863730353049 ) ) ;
#53692=CARTESIAN_POINT ( 'NONE',  ( -13.83322559834489418, 103.7219465388319577, 43.99456462701717641 ) ) ;
#53931=ORIENTED_EDGE ( 'NONE', *, *, #33889, .F. ) ;
#54184=CARTESIAN_POINT ( 'NONE',  ( -14.99731640896322027, 102.3427396610899365, 44.36017770743280408 ) ) ;
#54513=EDGE_CURVE ( 'NONE', #28157, #43464, #84243, .T. ) ;
#54546=AXIS2_PLACEMENT_3D ( 'NONE', #30574, #69064, #44268 ) ;
#54564=LINE ( 'NONE', #9508, #24742 ) ;
#54682=PLANE ( 'NONE',  #83428 ) ;
#54850=CARTESIAN_POINT ( 'NONE',  ( -29.54910080626416047, 95.88061498994892418, 44.62839885622795322 ) ) ;
#54876=CARTESIAN_POINT ( 'NONE',  ( -13.93676304270635136, 104.6887507934693105, 43.89948692389422291 ) ) ;
#55077=( NAMED_UNIT ( * ) SI_UNIT ( $, .STERADIAN. ) SOLID_ANGLE_UNIT ( ) );
#55086=FACE_OUTER_BOUND ( 'NONE', #66640, .T. ) ;
#55136=B_SPLINE_CURVE_WITH_KNOTS ( 'NONE', 3,
 ( #91633, #53094, #22200, #98223, #21216, #28294, #14607, #45485, #91140, #4502, #83041, #36895, #29311, #35402, #59169, #60175, #97242, #90144, #21703, #83543, #89657, #82052, #14107, #28805, #13614, #20720, #67805, #98731, #22707, #78413, #47488 ),
 .UNSPECIFIED., .F., .F.,
 ( 4, 3, 3, 3, 3, 3, 3, 3, 3, 3, 4 ),
 ( 0.000000000000000000, 3.357709145156459696E-05, 6.715417940116844182E-05, 0.0001007313198657331928, 0.0001343084960840520677, 0.0001678856156954599166, 0.0002014626747008569686, 0.0002350397637044858380, 0.0002686169264846224240, 0.0003021940916574071827, 0.0003125816342522696090 ),
 .UNSPECIFIED. ) ;
#55276=ORIENTED_EDGE ( 'NONE', *, *, #31896, .F. ) ;
#55661=CARTESIAN_POINT ( 'NONE',  ( -15.31269525828471068, 104.2312461070085021, 36.50000000000000000 ) ) ;
#55678=FACE_BOUND ( 'NONE', #22670, .T. ) ;
#56034=DIRECTION ( 'NONE',  ( 1.000000000000000000, 0.000000000000000000, 0.000000000000000000 ) ) ;
#56450=UNCERTAINTY_MEASURE_WITH_UNIT (LENGTH_MEASURE( 1.000000000000000082E-05 ), #72094, 'distance_accuracy_value', 'NONE');
#56639=VERTEX_POINT ( 'NONE', #87424 ) ;
#56863=( NAMED_UNIT ( * ) SI_UNIT ( $, .STERADIAN. ) SOLID_ANGLE_UNIT ( ) );
#56947=DIRECTION ( 'NONE',  ( 0.5000000000000012212, -0.8660254037844380415, -0.000000000000000000 ) ) ;
#57169=CARTESIAN_POINT ( 'NONE',  ( -30.04356256989597185, 94.88921800892812541, 43.89948692389422291 ) ) ;
#57318=CARTESIAN_POINT ( 'NONE',  ( -32.86949478547433046, 94.43171332246730287, 43.89948692389422291 ) ) ;
#57349=AXIS2_PLACEMENT_3D ( 'NONE', #55661, #76982, #70899 ) ;
#57494=ORIENTED_EDGE ( 'NONE', *, *, #89379, .F. ) ;
#57543=PRODUCT_DEFINITION ( 'UNKNOWN', '', #91599, #63548 ) ;
#57572=CARTESIAN_POINT ( 'NONE',  ( -15.48667327915257452, 102.2334782771513630, 44.45097685414082633 ) ) ;
#58481=FACE_OUTER_BOUND ( 'NONE', #96438, .T. ) ;
#58527=ORIENTED_EDGE ( 'NONE', *, *, #10513, .F. ) ;
#58848=EDGE_LOOP ( 'NONE', ( #48958, #86221, #76260, #52635, #44355, #857 ) ) ;
#58964=ADVANCED_FACE ( 'NONE', ( #30762 ), #72247, .F. ) ;
#59005=CARTESIAN_POINT ( 'NONE',  ( -23.58050215487121548, 99.69631501643195293, 45.19940618238346275 ) ) ;
#59110=DIRECTION ( 'NONE',  ( -0.000000000000000000, -0.000000000000000000, 1.000000000000000000 ) ) ;
#59169=CARTESIAN_POINT ( 'NONE',  ( -20.82151326869808017, 95.08966588713798274, 45.19948828869558355 ) ) ;
#59476=VECTOR ( 'NONE', #31521, 1000.000000000000227 ) ;
#59511=CARTESIAN_POINT ( 'NONE',  ( -23.48760161379543732, 99.79357714821047409, 45.19946697165472216 ) ) ;
#59933=CYLINDRICAL_SURFACE ( 'NONE', #17441, 1.449999999999993072 ) ;
#60175=CARTESIAN_POINT ( 'NONE',  ( -20.81253355169515018, 95.09634674671917764, 45.19948544083312214 ) ) ;
#60206=LINE ( 'NONE', #21731, #72527 ) ;
#60435=CARTESIAN_POINT ( 'NONE',  ( -15.45538172674451616, 105.8574260514038627, 44.07251632651297513 ) ) ;
#60608=CARTESIAN_POINT ( 'NONE',  ( -32.96890249059735112, 94.81157474915079320, 43.92482684459560005 ) ) ;
#60941=CARTESIAN_POINT ( 'NONE',  ( -14.47810378888552130, 105.4554537110193024, 43.92042717844079647 ) ) ;
#60949=CARTESIAN_POINT ( 'NONE',  ( -30.57234814819119606, 96.78886779632826176, 44.55697900252199162 ) ) ;
#61005=CARTESIAN_POINT ( 'NONE',  ( -23.56280764616852963, 99.74919597147199113, 45.19946569820528737 ) ) ;
#61236=ORIENTED_EDGE ( 'NONE', *, *, #50440, .T. ) ;
#61361=ORIENTED_EDGE ( 'NONE', *, *, #17958, .T. ) ;
#61417=CIRCLE ( 'NONE', #17761, 1.449999999999993072 ) ;
#61451=CARTESIAN_POINT ( 'NONE',  ( -29.35832683651975472, 95.01536403814361620, 44.58472265727041872 ) ) ;
#61793=DIRECTION ( 'NONE',  ( 0.000000000000000000, -0.000000000000000000, 1.000000000000000000 ) ) ;
#61938=CARTESIAN_POINT ( 'NONE',  ( -29.35927996735550494, 95.14472354011699906, 44.59528332425108488 ) ) ;
#62292=FACE_OUTER_BOUND ( 'NONE', #91313, .T. ) ;
#62347=VERTEX_POINT ( 'NONE', #28949 ) ;
#62389=ORIENTED_EDGE ( 'NONE', *, *, #70720, .F. ) ;
#62395=AXIS2_PLACEMENT_3D ( 'NONE', #25945, #11254, #26439 ) ;
#62665=MECHANICAL_DESIGN_GEOMETRIC_PRESENTATION_REPRESENTATION('',(#98349),#1224);
#62798=CARTESIAN_POINT ( 'NONE',  ( -14.12737304691700402, 103.0317842862404518, 44.13135102960670508 ) ) ;
#62910=EDGE_CURVE ( 'NONE', #67256, #34021, #30274, .T. ) ;
#63225=CARTESIAN_POINT ( 'NONE',  ( -32.94356256989595977, 94.88921800892812541, 36.50000000000000000 ) ) ;
#63485=CARTESIAN_POINT ( 'NONE',  ( -13.82959147685579104, 104.2312461070085021, 43.93259070532315036 ) ) ;
#63497=VERTEX_POINT ( 'NONE', #75451 ) ;
#63548=PRODUCT_DEFINITION_CONTEXT ( 'detailed design', #5180, 'design' ) ;
#63681=EDGE_CURVE ( 'NONE', #18286, #67256, #19161, .T. ) ;
#64105=DIRECTION ( 'NONE',  ( 0.000000000000000000, -0.000000000000000000, 1.000000000000000000 ) ) ;
#64344=EDGE_LOOP ( 'NONE', ( #37111, #35866, #33998, #16389 ) ) ;
#64873=VERTEX_POINT ( 'NONE', #37091 ) ;
#65155=CARTESIAN_POINT ( 'NONE',  ( -31.49356256989596758, 94.88921800892812541, 36.50000000000000000 ) ) ;
#65396=ORIENTED_EDGE ( 'NONE', *, *, #41544, .F. ) ;
#65583=DIRECTION ( 'NONE',  ( -0.000000000000000000, -0.000000000000000000, 1.000000000000000000 ) ) ;
#65729=VECTOR ( 'NONE', #6701, 999.9999999999998863 ) ;
#65930=EDGE_LOOP ( 'NONE', ( #77366, #8132, #83591, #61236 ) ) ;
#66148=ORIENTED_EDGE ( 'NONE', *, *, #70720, .T. ) ;
#66248=CARTESIAN_POINT ( 'NONE',  ( -15.31269525828471068, 104.2312461070085021, 45.19948692389422717 ) ) ;
#66640=EDGE_LOOP ( 'NONE', ( #3766, #19559, #67115 ) ) ;
#66836=AXIS2_PLACEMENT_3D ( 'NONE', #75211, #21018, #89454 ) ;
#66956=DIRECTION ( 'NONE',  ( -0.8660254037844378194, -0.5000000000000013323, -0.000000000000000000 ) ) ;
#67115=ORIENTED_EDGE ( 'NONE', *, *, #72157, .F. ) ;
#67125=CARTESIAN_POINT ( 'NONE',  ( -23.57381662850335147, 99.72943373905189901, 45.19944339805625333 ) ) ;
#67129=EDGE_CURVE ( 'NONE', #32333, #30740, #81289, .T. ) ;
#67256=VERTEX_POINT ( 'NONE', #57169 ) ;
#67422=ORIENTED_EDGE ( 'NONE', *, *, #11483, .F. ) ;
#67459=DIRECTION ( 'NONE',  ( 1.000000000000000000, 0.000000000000000000, 0.000000000000000000 ) ) ;
#67539=DIRECTION ( 'NONE',  ( 1.000000000000000000, 0.000000000000000000, 0.000000000000000000 ) ) ;
#67571=DIRECTION ( 'NONE',  ( 1.000000000000000000, 0.000000000000000000, 0.000000000000000000 ) ) ;
#67624=CARTESIAN_POINT ( 'NONE',  ( -23.44353372814872216, 99.78638950773219563, 45.19941947175312436 ) ) ;
#67805=CARTESIAN_POINT ( 'NONE',  ( -20.77630098335523812, 95.20697321020988113, 45.19938011207119644 ) ) ;
#68054=CARTESIAN_POINT ( 'NONE',  ( -16.91593106145283087, 105.3412939927731173, 44.39172944529203590 ) ) ;
#68061=CARTESIAN_POINT ( 'NONE',  ( -32.35580655284284290, 96.47003284356902952, 44.23339904099978526 ) ) ;
#68121=CARTESIAN_POINT ( 'NONE',  ( -23.56652710931154360, 99.64324603395651536, 45.19937630303415688 ) ) ;
#68250=DIRECTION ( 'NONE',  ( -0.000000000000000000, -0.000000000000000000, 1.000000000000000000 ) ) ;
#68427=FACE_OUTER_BOUND ( 'NONE', #99651, .T. ) ;
#68556=CARTESIAN_POINT ( 'NONE',  ( -31.69055000258023824, 96.81751122025097800, 44.38391476979933969 ) ) ;
#68618=CARTESIAN_POINT ( 'NONE',  ( -23.52037902133706027, 99.78538021036720806, 45.19948689642177442 ) ) ;
#68784=AXIS2_PLACEMENT_3D ( 'NONE', #15354, #91924, #23457 ) ;
#68875=CARTESIAN_POINT ( 'NONE',  ( -31.86539417309037958, 93.39048508798869364, 43.98374761209485229 ) ) ;
#68886=AXIS2_PLACEMENT_3D ( 'NONE', #17416, #87893, #25526 ) ;
#69064=DIRECTION ( 'NONE',  ( -0.000000000000000000, -0.000000000000000000, 1.000000000000000000 ) ) ;
#69082=CARTESIAN_POINT ( 'NONE',  ( -13.88625461359388957, 104.5404930901994334, 43.90693181722170380 ) ) ;
#69136=EDGE_CURVE ( 'NONE', #34021, #91664, #30179, .T. ) ;
#69536=CARTESIAN_POINT ( 'NONE',  ( -42.74117156905490589, 79.73515388767964396, 36.50000000000000000 ) ) ;
#69558=CARTESIAN_POINT ( 'NONE',  ( -32.15221709332305977, 96.62083620615463531, 44.28563379145492007 ) ) ;
#69892=DIRECTION ( 'NONE',  ( -0.000000000000000000, -0.000000000000000000, 1.000000000000000000 ) ) ;
#69899=CARTESIAN_POINT ( 'NONE',  ( -14.00244190342910144, 103.2482637300012698, 44.08288450968263561 ) ) ;
#70158=B_SPLINE_CURVE_WITH_KNOTS ( 'NONE', 3,
 ( #87803, #10739, #81175, #57318 ),
 .UNSPECIFIED., .F., .F.,
 ( 4, 4 ),
 ( 1.962615573354718958E-17, 0.0005839710162101796522 ),
 .UNSPECIFIED. ) ;
#70280=DIRECTION ( 'NONE',  ( -0.000000000000000000, -0.000000000000000000, 1.000000000000000000 ) ) ;
#70364=ORIENTED_EDGE ( 'NONE', *, *, #17040, .T. ) ;
#70444=( GEOMETRIC_REPRESENTATION_CONTEXT ( 3 ) GLOBAL_UNCERTAINTY_ASSIGNED_CONTEXT ( ( #56450 ) ) GLOBAL_UNIT_ASSIGNED_CONTEXT ( ( #72094, #78695, #56863 ) ) REPRESENTATION_CONTEXT ( 'NONE', 'WORKASPACE' ) );
#70720=EDGE_CURVE ( 'NONE', #62347, #100289, #37420, .T. ) ;
#70741=DIRECTION ( 'NONE',  ( -0.000000000000000000, -0.000000000000000000, 1.000000000000000000 ) ) ;
#70899=DIRECTION ( 'NONE',  ( 1.000000000000000000, 0.000000000000000000, 0.000000000000000000 ) ) ;
#70922=CARTESIAN_POINT ( 'NONE',  ( -15.11550709823832861, 102.3030086117089752, 44.38387608498982928 ) ) ;
#71098=SHAPE_REPRESENTATION_RELATIONSHIP ( 'NONE' , 'NONE' ,  #77412, #29552 ) ;
#71755=LINE ( 'NONE', #40809, #73513 ) ;
#72094=( LENGTH_UNIT ( ) NAMED_UNIT ( * ) SI_UNIT ( .MILLI., .METRE. ) );
#72157=EDGE_CURVE ( 'NONE', #82522, #56639, #95258, .T. ) ;
#72176=ORIENTED_EDGE ( 'NONE', *, *, #73839, .T. ) ;
#72247=CONICAL_SURFACE ( 'NONE', #33391, 2.749999999999999112, 0.7853981633974469467 ) ;
#72414=ADVANCED_FACE ( 'NONE', ( #68427 ), #91770, .T. ) ;
#72527=VECTOR ( 'NONE', #91166, 1000.000000000000000 ) ;
#72674=ORIENTED_EDGE ( 'NONE', *, *, #20094, .F. ) ;
#72706=AXIS2_PLACEMENT_3D ( 'NONE', #30069, #4801, #67571 ) ;
#72785=CIRCLE ( 'NONE', #89029, 1.449999999999993072 ) ;
#72902=ORIENTED_EDGE ( 'NONE', *, *, #54513, .F. ) ;
#72966=ADVANCED_FACE ( 'NONE', ( #90436 ), #14500, .F. ) ;
#73513=VECTOR ( 'NONE', #41823, 1000.000000000000000 ) ;
#73610=AXIS2_PLACEMENT_3D ( 'NONE', #88091, #79473, #49033 ) ;
#73670=CARTESIAN_POINT ( 'NONE',  ( -27.23973145446879940, 106.0054225863516280, 45.19937630303415688 ) ) ;
#73696=DIRECTION ( 'NONE',  ( 1.000000000000000000, 0.000000000000000000, 0.000000000000000000 ) ) ;
#73839=EDGE_CURVE ( 'NONE', #34021, #63497, #61417, .T. ) ;
#73855=AXIS2_PLACEMENT_3D ( 'NONE', #86073, #92640, #16597 ) ;
#73905=AXIS2_PLACEMENT_3D ( 'NONE', #65155, #18072, #56034 ) ;
#74095=EDGE_LOOP ( 'NONE', ( #84964, #24327, #19275, #17632 ) ) ;
#74132=EDGE_CURVE ( 'NONE', #52552, #87881, #17603, .T. ) ;
#74414=CARTESIAN_POINT ( 'NONE',  ( -23.39332202855467813, 99.74324603395649547, 45.19937630303414977 ) ) ;
#74444=DIRECTION ( 'NONE',  ( -0.7071067811865465735, 8.659560562354921765E-17, 0.7071067811865484609 ) ) ;
#75211=CARTESIAN_POINT ( 'NONE',  ( -27.15312891409035601, 106.0554225863516109, 0.000000000000000000 ) ) ;
#75451=CARTESIAN_POINT ( 'NONE',  ( -32.86949478547433046, 94.43171332246730287, 43.89948692389422291 ) ) ;
#75610=CARTESIAN_POINT ( 'NONE',  ( -4.065086259125790136, 119.3853102282570120, 36.50000000000000000 ) ) ;
#75638=CIRCLE ( 'NONE', #82184, 1.449999999999994627 ) ;
#75673=CARTESIAN_POINT ( 'NONE',  ( -15.98639401305193175, 105.8318875400968011, 44.17750287558818911 ) ) ;
#75748=CARTESIAN_POINT ( 'NONE',  ( -23.57584832053852963, 99.66285025437392164, 45.19938011207119644 ) ) ;
#75790=EDGE_CURVE ( 'NONE', #1578, #62347, #75638, .T. ) ;
#75938=EDGE_CURVE ( 'NONE', #43464, #4742, #22929, .T. ) ;
#76024=CARTESIAN_POINT ( 'NONE',  ( -29.37075727991403440, 94.88921800892813962, 44.57229221387616036 ) ) ;
#76089=SHAPE_DEFINITION_REPRESENTATION ( #82432, #77412 ) ;
#76252=CARTESIAN_POINT ( 'NONE',  ( -23.57130163085902552, 99.65262297949493586, 45.19937752447436452 ) ) ;
#76260=ORIENTED_EDGE ( 'NONE', *, *, #46988, .T. ) ;
#76280=ORIENTED_EDGE ( 'NONE', *, *, #12128, .F. ) ;
#76283=DIRECTION ( 'NONE',  ( -0.5000000000000012212, 0.8660254037844380415, 0.000000000000000000 ) ) ;
#76389=MANIFOLD_SOLID_BREP ( 'Split Line2', #36149 ) ;
#76756=LINE ( 'NONE', #38745, #98219 ) ;
#76926=CARTESIAN_POINT ( 'NONE',  ( -12.56269525828471245, 104.2312461070085021, 45.19948692389422717 ) ) ;
#76982=DIRECTION ( 'NONE',  ( 0.000000000000000000, -0.000000000000000000, 1.000000000000000000 ) ) ;
#77159=CARTESIAN_POINT ( 'NONE',  ( -30.22909824404765899, 96.62485709217924068, 44.59310059583850716 ) ) ;
#77202=CIRCLE ( 'NONE', #90192, 1.449999999999994627 ) ;
#77366=ORIENTED_EDGE ( 'NONE', *, *, #88200, .T. ) ;
#77412=SHAPE_REPRESENTATION ( 'Circular Angle Protractor Plate', ( #68784 ), #70444 ) ;
#77522=CARTESIAN_POINT ( 'NONE',  ( -15.31269525828471068, 104.2312461070085021, 43.89948692389422291 ) ) ;
#77527=ORIENTED_EDGE ( 'NONE', *, *, #46988, .F. ) ;
#77826=DIRECTION ( 'NONE',  ( 1.000000000000000000, 0.000000000000000000, 0.000000000000000000 ) ) ;
#77861=CARTESIAN_POINT ( 'NONE',  ( -50.24117156905492720, 92.72553494444620981, 36.50000000000000000 ) ) ;
#78121=CONICAL_SURFACE ( 'NONE', #21421, 2.749999999999999112, 0.7853981633974469467 ) ;
#78413=CARTESIAN_POINT ( 'NONE',  ( -20.78386844332395711, 95.22353984434415963, 45.19937630303414977 ) ) ;
#78527=CARTESIAN_POINT ( 'NONE',  ( -17.43550054826663498, 104.2312461070085021, 44.57229221387615326 ) ) ;
#78695=( NAMED_UNIT ( * ) PLANE_ANGLE_UNIT ( ) SI_UNIT ( $, .RADIAN. ) );
#78864=DIRECTION ( 'NONE',  ( 1.000000000000000000, 0.000000000000000000, 0.000000000000000000 ) ) ;
#79473=DIRECTION ( 'NONE',  ( -0.5000000000000013323, 0.8660254037844380415, -0.000000000000000000 ) ) ;
#79814=ORIENTED_EDGE ( 'NONE', *, *, #69136, .F. ) ;
#80039=EDGE_CURVE ( 'NONE', #30740, #67256, #11221, .T. ) ;
#80434=CARTESIAN_POINT ( 'NONE',  ( -17.05341241735402136, 102.9187400387798874, 44.62585372971393127 ) ) ;
#81175=CARTESIAN_POINT ( 'NONE',  ( -32.80726662848048392, 94.24456392606165878, 43.88975813191157016 ) ) ;
#81289=B_SPLINE_CURVE_WITH_KNOTS ( 'NONE', 3,
 ( #76024, #5598, #37474, #85647, #47082, #30889, #86154, #93733, #992, #31872, #92724, #23779, #15676, #68875, #46571, #24778, #92244, #85128 ),
 .UNSPECIFIED., .F., .F.,
 ( 4, 2, 2, 2, 2, 2, 2, 2, 4 ),
 ( 0.006884441260529831907, 0.007422657591717915157, 0.007960873922905998407, 0.008499090254094083391, 0.009037306585282166640, 0.009575522916470241216, 0.01011373924765832447, 0.01065195557884640945, 0.01119017191003449270 ),
 .UNSPECIFIED. ) ;
#81362=DIRECTION ( 'NONE',  ( 1.000000000000000000, 0.000000000000000000, 0.000000000000000000 ) ) ;
#81464=DIRECTION ( 'NONE',  ( 0.8660254037844378194, 0.5000000000000014433, 0.000000000000000000 ) ) ;
#81608=ORIENTED_EDGE ( 'NONE', *, *, #74132, .T. ) ;
#82052=CARTESIAN_POINT ( 'NONE',  ( -20.77549415122608067, 95.15121615758417306, 45.19943101769310090 ) ) ;
#82135=ORIENTED_EDGE ( 'NONE', *, *, #69136, .T. ) ;
#82184=AXIS2_PLACEMENT_3D ( 'NONE', #43235, #51340, #67539 ) ;
#82340=DIRECTION ( 'NONE',  ( 1.000000000000000000, 0.000000000000000000, 0.000000000000000000 ) ) ;
#82432=PRODUCT_DEFINITION_SHAPE ( 'NONE', 'NONE',  #57543 ) ;
#82522=VERTEX_POINT ( 'NONE', #15209 ) ;
#82720=DIRECTION ( 'NONE',  ( -0.000000000000000000, -0.000000000000000000, 1.000000000000000000 ) ) ;
#82982=ORIENTED_EDGE ( 'NONE', *, *, #48490, .T. ) ;
#83041=CARTESIAN_POINT ( 'NONE',  ( -20.86454769009831978, 95.07624631637331447, 45.19946697165472216 ) ) ;
#83283=DIRECTION ( 'NONE',  ( -0.000000000000000000, -0.000000000000000000, 1.000000000000000000 ) ) ;
#83321=CARTESIAN_POINT ( 'NONE',  ( -13.82959147685579104, 104.2312461070085021, 43.93259070532315036 ) ) ;
#83366=CARTESIAN_POINT ( 'NONE',  ( -23.39891821046326825, 99.75293890535058949, 45.19937630303414977 ) ) ;
#83428=AXIS2_PLACEMENT_3D ( 'NONE', #46590, #61793, #9631 ) ;
#83543=CARTESIAN_POINT ( 'NONE',  ( -20.78307953964266019, 95.12990406498558116, 45.19945594742419104 ) ) ;
#83591=ORIENTED_EDGE ( 'NONE', *, *, #72157, .T. ) ;
#83624=CIRCLE ( 'NONE', #73905, 1.449999999999993072 ) ;
#83871=VECTOR ( 'NONE', #56947, 999.9999999999998863 ) ;
#84005=ORIENTED_EDGE ( 'NONE', *, *, #80039, .F. ) ;
#84243=LINE ( 'NONE', #75610, #65729 ) ;
#84300=CARTESIAN_POINT ( 'NONE',  ( -16.32499242613253543, 105.7308263295076216, 44.25048734575928222 ) ) ;
#84692=PRODUCT_CONTEXT ( 'NONE', #51809, 'mechanical' ) ;
#84964=ORIENTED_EDGE ( 'NONE', *, *, #17958, .F. ) ;
#85128=CARTESIAN_POINT ( 'NONE',  ( -32.57773935851065517, 93.92637809958223727, 43.89948692389421581 ) ) ;
#85647=CARTESIAN_POINT ( 'NONE',  ( -29.57042460543627982, 94.20560631922556638, 44.48281236311225939 ) ) ;
#85922=UNCERTAINTY_MEASURE_WITH_UNIT (LENGTH_MEASURE( 1.000000000000000082E-05 ), #100216, 'distance_accuracy_value', 'NONE');
#86048=CARTESIAN_POINT ( 'NONE',  ( -20.95882727533908252, 95.12657743062730731, 45.19937630303415688 ) ) ;
#86062=CARTESIAN_POINT ( 'NONE',  ( -16.76269525828470464, 104.2312461070085021, 45.19948692389422717 ) ) ;
#86073=CARTESIAN_POINT ( 'NONE',  ( -15.31269525828471068, 104.2312461070085021, 45.19948692389422717 ) ) ;
#86097=CARTESIAN_POINT ( 'NONE',  ( -20.78562219458220284, 95.22657743062728741, 45.19937630303414267 ) ) ;
#86154=CARTESIAN_POINT ( 'NONE',  ( -30.02241387713131004, 93.66080434060147297, 44.35815572581725519 ) ) ;
#86221=ORIENTED_EDGE ( 'NONE', *, *, #46075, .F. ) ;
#86310=CARTESIAN_POINT ( 'NONE',  ( -31.49356256989596758, 94.88921800892812541, 45.19948692389422717 ) ) ;
#86467=CARTESIAN_POINT ( 'NONE',  ( -23.56652710931154360, 99.64324603395651536, 45.19937630303415688 ) ) ;
#86695=AXIS2_PLACEMENT_3D ( 'NONE', #66248, #59110, #36329 ) ;
#86815=DIRECTION ( 'NONE',  ( -0.000000000000000000, -0.000000000000000000, 1.000000000000000000 ) ) ;
#86869=CARTESIAN_POINT ( 'NONE',  ( -32.95600942927097066, 94.73368306973679864, 43.91807046316925778 ) ) ;
#87127=ORIENTED_EDGE ( 'NONE', *, *, #48490, .F. ) ;
#87369=CIRCLE ( 'NONE', #72706, 1.449999999999993072 ) ;
#87424=CARTESIAN_POINT ( 'NONE',  ( -14.22851846967002487, 105.1940860163543476, 43.89948692389422291 ) ) ;
#87803=CARTESIAN_POINT ( 'NONE',  ( -32.57773935851065517, 93.92637809958223727, 43.89948692389421581 ) ) ;
#87881=VERTEX_POINT ( 'NONE', #86467 ) ;
#87893=DIRECTION ( 'NONE',  ( -0.000000000000000000, -0.000000000000000000, 1.000000000000000000 ) ) ;
#88091=CARTESIAN_POINT ( 'NONE',  ( -19.65312891409034179, 93.06504152958504505, 0.000000000000000000 ) ) ;
#88200=EDGE_CURVE ( 'NONE', #4089, #100289, #4404, .T. ) ;
#88545=CARTESIAN_POINT ( 'NONE',  ( -15.35952475613307655, 102.2482863741581980, 44.42918405269885795 ) ) ;
#89029=AXIS2_PLACEMENT_3D ( 'NONE', #33206, #64105, #77826 ) ;
#89189=CARTESIAN_POINT ( 'NONE',  ( -34.24356256989597114, 94.88921800892812541, 45.19948692389422717 ) ) ;
#89379=EDGE_CURVE ( 'NONE', #63497, #91664, #634, .T. ) ;
#89454=DIRECTION ( 'NONE',  ( 0.8660254037844378194, 0.5000000000000014433, 0.000000000000000000 ) ) ;
#89577=CYLINDRICAL_SURFACE ( 'NONE', #18176, 45.19948692389423428 ) ;
#89657=CARTESIAN_POINT ( 'NONE',  ( -20.77833267539040918, 95.14038972553191797, 45.19944339805625333 ) ) ;
#89719=EDGE_LOOP ( 'NONE', ( #17526, #76280, #26378, #20164 ) ) ;
#89838=CIRCLE ( 'NONE', #73610, 45.19948692389423428 ) ;
#90144=CARTESIAN_POINT ( 'NONE',  ( -20.79560377010869487, 95.11135092968059723, 45.19947544897750191 ) ) ;
#90192=AXIS2_PLACEMENT_3D ( 'NONE', #93766, #31905, #24324 ) ;
#90436=FACE_OUTER_BOUND ( 'NONE', #14574, .T. ) ;
#90626=ORIENTED_EDGE ( 'NONE', *, *, #62910, .F. ) ;
#90914=CARTESIAN_POINT ( 'NONE',  ( -17.41797074981450777, 104.4091411665443871, 44.55476241542402960 ) ) ;
#90978=CARTESIAN_POINT ( 'NONE',  ( -23.39332202855467813, 99.74324603395649547, 45.19937630303414977 ) ) ;
#91101=CARTESIAN_POINT ( 'NONE',  ( -31.49356256989596758, 94.88921800892812541, 45.19948692389422717 ) ) ;
#91140=CARTESIAN_POINT ( 'NONE',  ( -20.88691866978057377, 95.07703167464532612, 45.19944471151773513 ) ) ;
#91166=DIRECTION ( 'NONE',  ( -0.7071067811865462405, 8.659560562354915602E-17, 0.7071067811865489050 ) ) ;
#91313=EDGE_LOOP ( 'NONE', ( #67422, #14548, #52124, #77527 ) ) ;
#91461=CARTESIAN_POINT ( 'NONE',  ( -23.55654553378506932, 99.75847253490320554, 45.19947544897750191 ) ) ;
#91599=PRODUCT_DEFINITION_FORMATION_WITH_SPECIFIED_SOURCE ( 'ANY', '', #26520, .NOT_KNOWN. ) ;
#91633=CARTESIAN_POINT ( 'NONE',  ( -20.95882727533908252, 95.12657743062730731, 45.19937630303415688 ) ) ;
#91664=VERTEX_POINT ( 'NONE', #22689 ) ;
#91770=PLANE ( 'NONE',  #8007 ) ;
#91907=CARTESIAN_POINT ( 'NONE',  ( -30.02137776312446960, 96.47624038658500467, 44.61044380647359731 ) ) ;
#91924=DIRECTION ( 'NONE',  ( 0.000000000000000000, 0.000000000000000000, 1.000000000000000000 ) ) ;
#92169=CONICAL_SURFACE ( 'NONE', #30661, 2.749999999999999112, 0.7853981633974463916 ) ;
#92176=CARTESIAN_POINT ( 'NONE',  ( -14.09755945733355276, 105.0466235773165096, 43.88975835780059498 ) ) ;
#92244=CARTESIAN_POINT ( 'NONE',  ( -32.46306855948172654, 93.78642701249712843, 43.90667800897207940 ) ) ;
#92263=CARTESIAN_POINT ( 'NONE',  ( -13.82959147685579104, 104.2312461070085021, 43.93259070532315036 ) ) ;
#92395=CARTESIAN_POINT ( 'NONE',  ( -14.77590589997254611, 105.6530250111700013, 43.95880336568158242 ) ) ;
#92402=CARTESIAN_POINT ( 'NONE',  ( -29.37075727991403440, 94.88921800892813962, 44.57229221387616036 ) ) ;
#92640=DIRECTION ( 'NONE',  ( -0.000000000000000000, -0.000000000000000000, 1.000000000000000000 ) ) ;
#92724=CARTESIAN_POINT ( 'NONE',  ( -30.99490618150352006, 93.26309149566453982, 44.14155221573258103 ) ) ;
#92914=CARTESIAN_POINT ( 'NONE',  ( -13.85019419761653836, 104.3865186021088078, 43.91809099165308083 ) ) ;
#93154=AXIS2_PLACEMENT_3D ( 'NONE', #52559, #53067, #13586 ) ;
#93158=FACE_OUTER_BOUND ( 'NONE', #22804, .T. ) ;
#93242=CARTESIAN_POINT ( 'NONE',  ( -14.65437209019651732, 102.4994735386711397, 44.28570614930890059 ) ) ;
#93397=CARTESIAN_POINT ( 'NONE',  ( -31.80880183691780871, 96.77778971401760089, 44.36020821963600724 ) ) ;
#93426=CARTESIAN_POINT ( 'NONE',  ( -13.83735209449856640, 104.3088569339948180, 43.92483008768037678 ) ) ;
#93461=FACE_OUTER_BOUND ( 'NONE', #37147, .T. ) ;
#93569=CARTESIAN_POINT ( 'NONE',  ( 3.434913740874227628, 106.3949291714904462, 36.50000000000000000 ) ) ;
#93630=DIRECTION ( 'NONE',  ( 0.5000000000000012212, -0.8660254037844380415, -0.000000000000000000 ) ) ;
#93733=CARTESIAN_POINT ( 'NONE',  ( -30.31876249839593385, 93.46524241893469309, 44.28731163467956833 ) ) ;
#93752=FACE_OUTER_BOUND ( 'NONE', #89719, .T. ) ;
#93754=CARTESIAN_POINT ( 'NONE',  ( -16.79610892523035659, 102.6363712329456916, 44.61266935656895072 ) ) ;
#93766=CARTESIAN_POINT ( 'NONE',  ( -15.31269525828471068, 104.2312461070085021, 43.89948692389422291 ) ) ;
#93783=ADVANCED_FACE ( 'NONE', ( #58481 ), #27615, .T. ) ;
#94103=EDGE_LOOP ( 'NONE', ( #98896, #66148, #33646 ) ) ;
#94248=CARTESIAN_POINT ( 'NONE',  ( -17.12851661768869604, 103.0207181397640284, 44.62810345821594638 ) ) ;
#94973=VERTEX_POINT ( 'NONE', #34594 ) ;
#95182=DIRECTION ( 'NONE',  ( -0.000000000000000000, -0.000000000000000000, 1.000000000000000000 ) ) ;
#95256=AXIS2_PLACEMENT_3D ( 'NONE', #77522, #69892, #99324 ) ;
#95258=B_SPLINE_CURVE_WITH_KNOTS ( 'NONE', 3,
 ( #35666, #90914, #46227, #31044, #21463, #68054, #38646, #21955, #84300, #75673, #52351, #60435, #14848, #99974, #92395, #60941, #45734, #30559 ),
 .UNSPECIFIED., .F., .F.,
 ( 4, 2, 2, 2, 2, 2, 2, 2, 4 ),
 ( 0.001647475917812264148, 0.002184538663664093924, 0.002721601409515923917, 0.003258664155367753910, 0.003795726901219583470, 0.004332789647071413029, 0.004869852392923247793, 0.005406915138775082556, 0.005943977884626917320 ),
 .UNSPECIFIED. ) ;
#95456=ORIENTED_EDGE ( 'NONE', *, *, #2059, .T. ) ;
#96438=EDGE_LOOP ( 'NONE', ( #49339, #61361, #70364, #81608 ) ) ;
#96530=FACE_OUTER_BOUND ( 'NONE', #94103, .T. ) ;
#96719=EDGE_LOOP ( 'NONE', ( #82982, #2273 ) ) ;
#96840=CIRCLE ( 'NONE', #95256, 1.449999999999994627 ) ;
#96901=CARTESIAN_POINT ( 'NONE',  ( -42.74117156905490589, 79.73515388767964396, 36.50000000000000000 ) ) ;
#96938=ORIENTED_EDGE ( 'NONE', *, *, #75938, .F. ) ;
#97242=CARTESIAN_POINT ( 'NONE',  ( -20.80355385027020176, 95.10302759471045420, 45.19948259297560611 ) ) ;
#97424=DIRECTION ( 'NONE',  ( -0.000000000000000000, -0.000000000000000000, 1.000000000000000000 ) ) ;
#97554=EDGE_CURVE ( 'NONE', #3234, #34021, #71755, .T. ) ;
#98049=CARTESIAN_POINT ( 'NONE',  ( -23.57959705543464324, 99.68515928958061068, 45.19939659820781230 ) ) ;
#98219=VECTOR ( 'NONE', #76283, 999.9999999999998863 ) ;
#98223=CARTESIAN_POINT ( 'NONE',  ( -20.93739514293010728, 95.10073009761491392, 45.19938842315524852 ) ) ;
#98308=AXIS2_PLACEMENT_3D ( 'NONE', #86310, #86815, #16845 ) ;
#98349=STYLED_ITEM('',(#100324),#76389);
#98726=CARTESIAN_POINT ( 'NONE',  ( -29.37075727991403440, 94.88921800892813962, 44.57229221387616036 ) ) ;
#98731=CARTESIAN_POINT ( 'NONE',  ( -20.78084767303474578, 95.21720048508885270, 45.19937752447436452 ) ) ;
#98896=ORIENTED_EDGE ( 'NONE', *, *, #30513, .F. ) ;
#98984=CARTESIAN_POINT ( 'NONE',  ( -29.67776128939880564, 96.09974013826338535, 44.62810019855511001 ) ) ;
#99049=CARTESIAN_POINT ( 'NONE',  ( -23.46523063411318688, 99.79279178993846244, 45.19944471151773513 ) ) ;
#99324=DIRECTION ( 'NONE',  ( 1.000000000000000000, 0.000000000000000000, 0.000000000000000000 ) ) ;
#99466=ORIENTED_EDGE ( 'NONE', *, *, #67129, .F. ) ;
#99482=CARTESIAN_POINT ( 'NONE',  ( -31.44664044020622384, 96.87218780021319731, 44.42919983564367925 ) ) ;
#99541=CARTESIAN_POINT ( 'NONE',  ( -23.56987677623957822, 99.64941792683403321, 45.19937671356586861 ) ) ;
#99651=EDGE_LOOP ( 'NONE', ( #65396, #96938 ) ) ;
#99974=CARTESIAN_POINT ( 'NONE',  ( -14.93908996228087993, 105.7294041250763712, 43.98345477057558384 ) ) ;
#100216=( LENGTH_UNIT ( ) NAMED_UNIT ( * ) SI_UNIT ( .MILLI., .METRE. ) );
#100289=VERTEX_POINT ( 'NONE', #83321 ) ;
#100318=COLOUR_RGB('Sky Blue',0.24,0.69,0.87);
#100319=FILL_AREA_STYLE_COLOUR('',#100318);
#100320=FILL_AREA_STYLE('',(#100319));
#100321=SURFACE_STYLE_FILL_AREA(#100320);
#100322=SURFACE_SIDE_STYLE('',(#100321));
#100323=SURFACE_STYLE_USAGE(.BOTH.,#100322);
#100324=PRESENTATION_STYLE_ASSIGNMENT((#100323));
ENDSEC;
END-ISO-10303-21;
